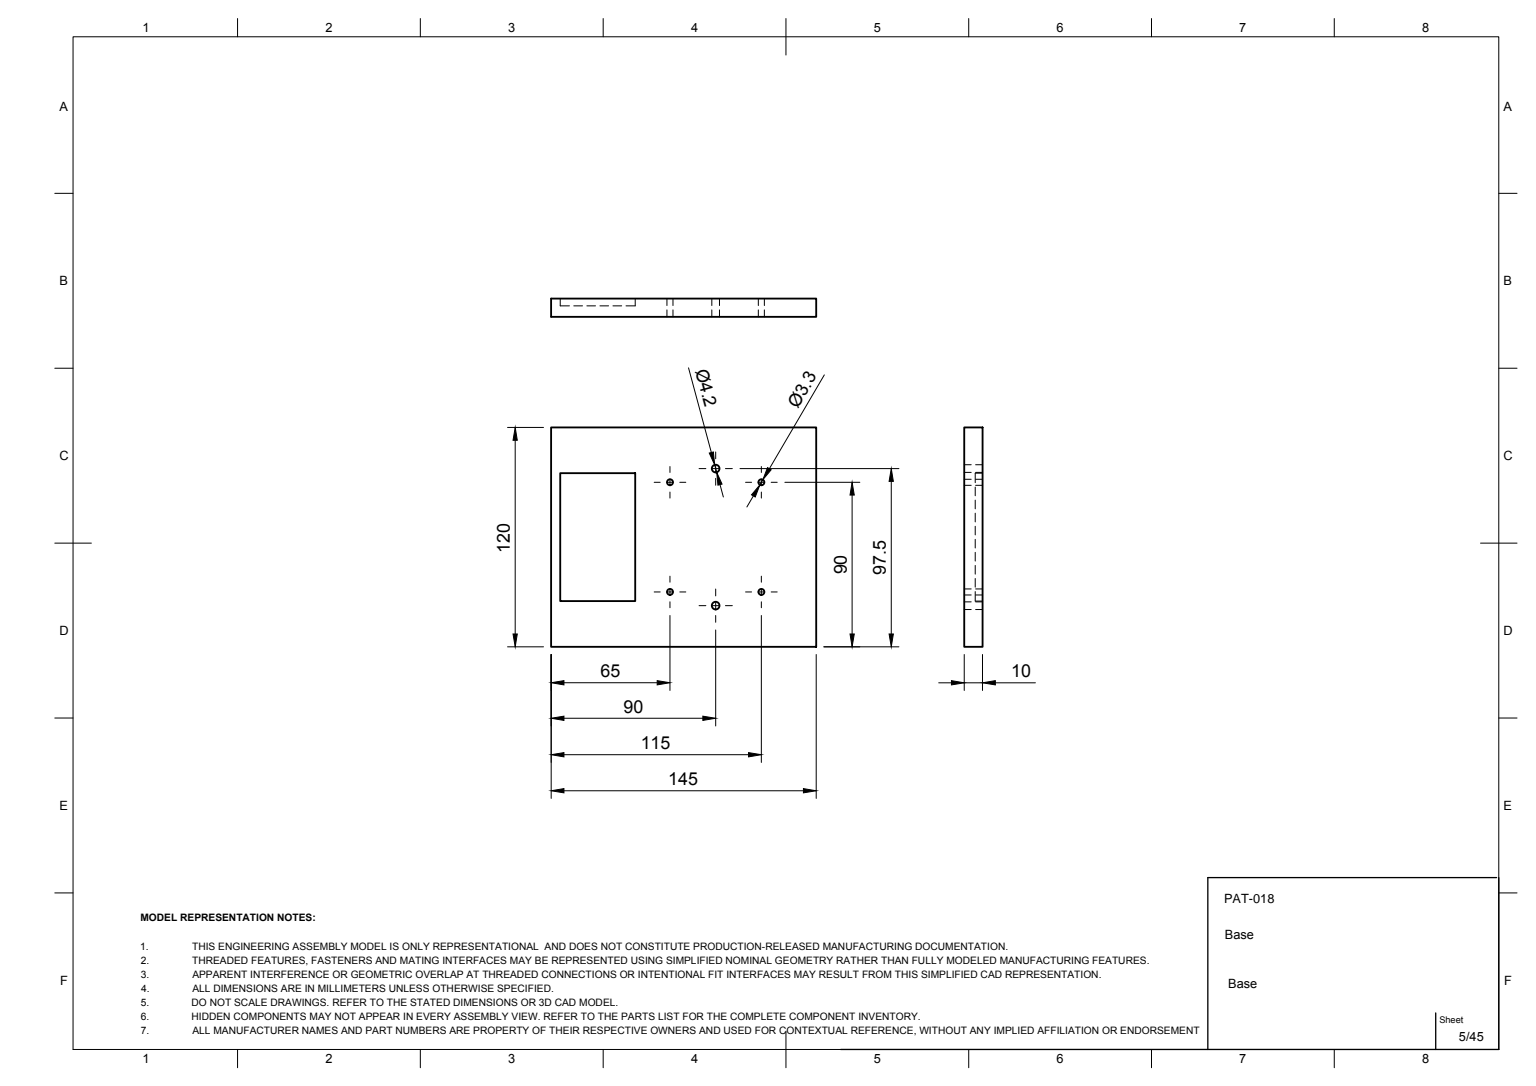
ISO-10303-21;
HEADER;
/* Generated by software containing ST-Developer
 * from STEP Tools, Inc. (www.steptools.com) 
 */

FILE_DESCRIPTION(
/* description */ ('Cam-driven reciprocating slide'),
/* implementation_level */ '2;1');

FILE_NAME(
/* name */ 'Base.step',
/* time_stamp */ '2026-10-28T03:25:20-07:00',
/* author */ (''),
/* organization */ (''),
/* preprocessor_version */ 'ST-DEVELOPER v20.2',
/* originating_system */ 'Autodesk Translation Framework v15.17.0.0',
/* authorisation */ '');

FILE_SCHEMA (('AUTOMOTIVE_DESIGN { 1 0 10303 214 3 1 1 }'));
ENDSEC;

DATA;
#10=MECHANICAL_DESIGN_GEOMETRIC_PRESENTATION_REPRESENTATION('',(#422),#13277);
#348=SHAPE_REPRESENTATION_RELATIONSHIP('SRR','None',#13441,#385);
#385=ADVANCED_BREP_SHAPE_REPRESENTATION('',(#466),#13236);
#422=STYLED_ITEM('',(#13699),#466);
#466=MANIFOLD_SOLID_BREP('Body1',#6398);
#507=FACE_BOUND('',#1296,.T.);
#508=FACE_BOUND('',#1297,.T.);
#509=FACE_BOUND('',#1298,.T.);
#510=FACE_BOUND('',#1299,.T.);
#511=FACE_BOUND('',#1300,.T.);
#512=FACE_BOUND('',#1301,.T.);
#513=FACE_BOUND('',#1302,.T.);
#514=FACE_BOUND('',#1304,.T.);
#515=FACE_BOUND('',#1305,.T.);
#516=FACE_BOUND('',#1306,.T.);
#517=FACE_BOUND('',#1307,.T.);
#518=FACE_BOUND('',#1308,.T.);
#519=FACE_BOUND('',#1309,.T.);
#681=PLANE('',#6874);
#682=PLANE('',#6875);
#683=PLANE('',#6876);
#684=PLANE('',#6877);
#685=PLANE('',#6878);
#686=PLANE('',#6879);
#687=PLANE('',#6880);
#688=PLANE('',#6881);
#689=PLANE('',#6882);
#690=PLANE('',#6883);
#691=PLANE('',#6884);
#901=FACE_OUTER_BOUND('',#1280,.T.);
#902=FACE_OUTER_BOUND('',#1281,.T.);
#903=FACE_OUTER_BOUND('',#1282,.T.);
#904=FACE_OUTER_BOUND('',#1283,.T.);
#905=FACE_OUTER_BOUND('',#1284,.T.);
#906=FACE_OUTER_BOUND('',#1285,.T.);
#907=FACE_OUTER_BOUND('',#1286,.T.);
#908=FACE_OUTER_BOUND('',#1287,.T.);
#909=FACE_OUTER_BOUND('',#1288,.T.);
#910=FACE_OUTER_BOUND('',#1289,.T.);
#911=FACE_OUTER_BOUND('',#1290,.T.);
#912=FACE_OUTER_BOUND('',#1291,.T.);
#913=FACE_OUTER_BOUND('',#1292,.T.);
#914=FACE_OUTER_BOUND('',#1293,.T.);
#915=FACE_OUTER_BOUND('',#1294,.T.);
#916=FACE_OUTER_BOUND('',#1295,.T.);
#917=FACE_OUTER_BOUND('',#1303,.T.);
#1280=EDGE_LOOP('',(#4336,#4337,#4338,#4339));
#1281=EDGE_LOOP('',(#4340,#4341,#4342,#4343));
#1282=EDGE_LOOP('',(#4344,#4345,#4346,#4347));
#1283=EDGE_LOOP('',(#4348,#4349,#4350,#4351));
#1284=EDGE_LOOP('',(#4352,#4353,#4354,#4355));
#1285=EDGE_LOOP('',(#4356,#4357,#4358,#4359));
#1286=EDGE_LOOP('',(#4360,#4361,#4362,#4363));
#1287=EDGE_LOOP('',(#4364,#4365,#4366,#4367));
#1288=EDGE_LOOP('',(#4368,#4369,#4370,#4371));
#1289=EDGE_LOOP('',(#4372,#4373,#4374,#4375));
#1290=EDGE_LOOP('',(#4376,#4377,#4378,#4379));
#1291=EDGE_LOOP('',(#4380,#4381,#4382,#4383));
#1292=EDGE_LOOP('',(#4384,#4385,#4386,#4387));
#1293=EDGE_LOOP('',(#4388,#4389,#4390,#4391));
#1294=EDGE_LOOP('',(#4392,#4393,#4394,#4395));
#1295=EDGE_LOOP('',(#4396,#4397,#4398,#4399));
#1296=EDGE_LOOP('',(#4400));
#1297=EDGE_LOOP('',(#4401));
#1298=EDGE_LOOP('',(#4402));
#1299=EDGE_LOOP('',(#4403));
#1300=EDGE_LOOP('',(#4404));
#1301=EDGE_LOOP('',(#4405));
#1302=EDGE_LOOP('',(#4406,#4407,#4408,#4409));
#1303=EDGE_LOOP('',(#4410,#4411,#4412,#4413));
#1304=EDGE_LOOP('',(#4414));
#1305=EDGE_LOOP('',(#4415));
#1306=EDGE_LOOP('',(#4416));
#1307=EDGE_LOOP('',(#4417));
#1308=EDGE_LOOP('',(#4418));
#1309=EDGE_LOOP('',(#4419));
#1833=LINE('',#9747,#2272);
#1834=LINE('',#9753,#2273);
#1835=LINE('',#9759,#2274);
#1836=LINE('',#9765,#2275);
#1837=LINE('',#9771,#2276);
#1838=LINE('',#9777,#2277);
#1839=LINE('',#9782,#2278);
#1840=LINE('',#9784,#2279);
#1841=LINE('',#9786,#2280);
#1842=LINE('',#9787,#2281);
#1843=LINE('',#9790,#2282);
#1844=LINE('',#9792,#2283);
#1845=LINE('',#9793,#2284);
#1846=LINE('',#9796,#2285);
#1847=LINE('',#9798,#2286);
#1848=LINE('',#9799,#2287);
#1849=LINE('',#9801,#2288);
#1850=LINE('',#9802,#2289);
#1851=LINE('',#9807,#2290);
#1852=LINE('',#9809,#2291);
#1853=LINE('',#9811,#2292);
#1854=LINE('',#9812,#2293);
#1855=LINE('',#9815,#2294);
#1856=LINE('',#9817,#2295);
#1857=LINE('',#9818,#2296);
#1858=LINE('',#9821,#2297);
#1859=LINE('',#9823,#2298);
#1860=LINE('',#9824,#2299);
#1861=LINE('',#9826,#2300);
#1862=LINE('',#9827,#2301);
#2272=VECTOR('',#7679,0.21);
#2273=VECTOR('',#7686,0.21);
#2274=VECTOR('',#7693,0.165);
#2275=VECTOR('',#7700,0.165);
#2276=VECTOR('',#7707,0.165);
#2277=VECTOR('',#7714,0.165);
#2278=VECTOR('',#7719,1.);
#2279=VECTOR('',#7720,1.);
#2280=VECTOR('',#7721,1.);
#2281=VECTOR('',#7722,1.);
#2282=VECTOR('',#7725,1.);
#2283=VECTOR('',#7726,1.);
#2284=VECTOR('',#7727,1.);
#2285=VECTOR('',#7730,1.);
#2286=VECTOR('',#7731,1.);
#2287=VECTOR('',#7732,1.);
#2288=VECTOR('',#7735,1.);
#2289=VECTOR('',#7736,1.);
#2290=VECTOR('',#7741,1.);
#2291=VECTOR('',#7742,1.);
#2292=VECTOR('',#7743,1.);
#2293=VECTOR('',#7744,1.);
#2294=VECTOR('',#7747,1.);
#2295=VECTOR('',#7748,1.);
#2296=VECTOR('',#7749,1.);
#2297=VECTOR('',#7752,1.);
#2298=VECTOR('',#7753,1.);
#2299=VECTOR('',#7754,1.);
#2300=VECTOR('',#7757,1.);
#2301=VECTOR('',#7758,1.);
#2711=CIRCLE('',#6857,0.21);
#2712=CIRCLE('',#6858,0.21);
#2713=CIRCLE('',#6860,0.21);
#2714=CIRCLE('',#6861,0.21);
#2715=CIRCLE('',#6863,0.165);
#2716=CIRCLE('',#6864,0.165);
#2717=CIRCLE('',#6866,0.165);
#2718=CIRCLE('',#6867,0.165);
#2719=CIRCLE('',#6869,0.165);
#2720=CIRCLE('',#6870,0.165);
#2721=CIRCLE('',#6872,0.165);
#2722=CIRCLE('',#6873,0.165);
#3035=VERTEX_POINT('',#9744);
#3036=VERTEX_POINT('',#9746);
#3037=VERTEX_POINT('',#9750);
#3038=VERTEX_POINT('',#9752);
#3039=VERTEX_POINT('',#9756);
#3040=VERTEX_POINT('',#9758);
#3041=VERTEX_POINT('',#9762);
#3042=VERTEX_POINT('',#9764);
#3043=VERTEX_POINT('',#9768);
#3044=VERTEX_POINT('',#9770);
#3045=VERTEX_POINT('',#9774);
#3046=VERTEX_POINT('',#9776);
#3047=VERTEX_POINT('',#9780);
#3048=VERTEX_POINT('',#9781);
#3049=VERTEX_POINT('',#9783);
#3050=VERTEX_POINT('',#9785);
#3051=VERTEX_POINT('',#9789);
#3052=VERTEX_POINT('',#9791);
#3053=VERTEX_POINT('',#9795);
#3054=VERTEX_POINT('',#9797);
#3055=VERTEX_POINT('',#9805);
#3056=VERTEX_POINT('',#9806);
#3057=VERTEX_POINT('',#9808);
#3058=VERTEX_POINT('',#9810);
#3059=VERTEX_POINT('',#9814);
#3060=VERTEX_POINT('',#9816);
#3061=VERTEX_POINT('',#9820);
#3062=VERTEX_POINT('',#9822);
#3558=EDGE_CURVE('',#3035,#3035,#2711,.T.);
#3559=EDGE_CURVE('',#3035,#3036,#1833,.T.);
#3560=EDGE_CURVE('',#3036,#3036,#2712,.T.);
#3561=EDGE_CURVE('',#3037,#3037,#2713,.T.);
#3562=EDGE_CURVE('',#3037,#3038,#1834,.T.);
#3563=EDGE_CURVE('',#3038,#3038,#2714,.T.);
#3564=EDGE_CURVE('',#3039,#3039,#2715,.T.);
#3565=EDGE_CURVE('',#3039,#3040,#1835,.T.);
#3566=EDGE_CURVE('',#3040,#3040,#2716,.T.);
#3567=EDGE_CURVE('',#3041,#3041,#2717,.T.);
#3568=EDGE_CURVE('',#3041,#3042,#1836,.T.);
#3569=EDGE_CURVE('',#3042,#3042,#2718,.T.);
#3570=EDGE_CURVE('',#3043,#3043,#2719,.T.);
#3571=EDGE_CURVE('',#3043,#3044,#1837,.T.);
#3572=EDGE_CURVE('',#3044,#3044,#2720,.T.);
#3573=EDGE_CURVE('',#3045,#3045,#2721,.T.);
#3574=EDGE_CURVE('',#3045,#3046,#1838,.T.);
#3575=EDGE_CURVE('',#3046,#3046,#2722,.T.);
#3576=EDGE_CURVE('',#3047,#3048,#1839,.T.);
#3577=EDGE_CURVE('',#3049,#3047,#1840,.T.);
#3578=EDGE_CURVE('',#3050,#3049,#1841,.T.);
#3579=EDGE_CURVE('',#3050,#3048,#1842,.T.);
#3580=EDGE_CURVE('',#3048,#3051,#1843,.T.);
#3581=EDGE_CURVE('',#3052,#3050,#1844,.T.);
#3582=EDGE_CURVE('',#3052,#3051,#1845,.T.);
#3583=EDGE_CURVE('',#3051,#3053,#1846,.T.);
#3584=EDGE_CURVE('',#3054,#3052,#1847,.T.);
#3585=EDGE_CURVE('',#3054,#3053,#1848,.T.);
#3586=EDGE_CURVE('',#3053,#3047,#1849,.T.);
#3587=EDGE_CURVE('',#3049,#3054,#1850,.T.);
#3588=EDGE_CURVE('',#3055,#3056,#1851,.T.);
#3589=EDGE_CURVE('',#3056,#3057,#1852,.T.);
#3590=EDGE_CURVE('',#3058,#3057,#1853,.T.);
#3591=EDGE_CURVE('',#3055,#3058,#1854,.T.);
#3592=EDGE_CURVE('',#3059,#3055,#1855,.T.);
#3593=EDGE_CURVE('',#3060,#3058,#1856,.T.);
#3594=EDGE_CURVE('',#3059,#3060,#1857,.T.);
#3595=EDGE_CURVE('',#3061,#3059,#1858,.T.);
#3596=EDGE_CURVE('',#3062,#3060,#1859,.T.);
#3597=EDGE_CURVE('',#3061,#3062,#1860,.T.);
#3598=EDGE_CURVE('',#3056,#3061,#1861,.T.);
#3599=EDGE_CURVE('',#3057,#3062,#1862,.T.);
#4336=ORIENTED_EDGE('',*,*,#3558,.F.);
#4337=ORIENTED_EDGE('',*,*,#3559,.T.);
#4338=ORIENTED_EDGE('',*,*,#3560,.F.);
#4339=ORIENTED_EDGE('',*,*,#3559,.F.);
#4340=ORIENTED_EDGE('',*,*,#3561,.F.);
#4341=ORIENTED_EDGE('',*,*,#3562,.T.);
#4342=ORIENTED_EDGE('',*,*,#3563,.F.);
#4343=ORIENTED_EDGE('',*,*,#3562,.F.);
#4344=ORIENTED_EDGE('',*,*,#3564,.F.);
#4345=ORIENTED_EDGE('',*,*,#3565,.T.);
#4346=ORIENTED_EDGE('',*,*,#3566,.F.);
#4347=ORIENTED_EDGE('',*,*,#3565,.F.);
#4348=ORIENTED_EDGE('',*,*,#3567,.F.);
#4349=ORIENTED_EDGE('',*,*,#3568,.T.);
#4350=ORIENTED_EDGE('',*,*,#3569,.F.);
#4351=ORIENTED_EDGE('',*,*,#3568,.F.);
#4352=ORIENTED_EDGE('',*,*,#3570,.F.);
#4353=ORIENTED_EDGE('',*,*,#3571,.T.);
#4354=ORIENTED_EDGE('',*,*,#3572,.F.);
#4355=ORIENTED_EDGE('',*,*,#3571,.F.);
#4356=ORIENTED_EDGE('',*,*,#3573,.F.);
#4357=ORIENTED_EDGE('',*,*,#3574,.T.);
#4358=ORIENTED_EDGE('',*,*,#3575,.F.);
#4359=ORIENTED_EDGE('',*,*,#3574,.F.);
#4360=ORIENTED_EDGE('',*,*,#3576,.F.);
#4361=ORIENTED_EDGE('',*,*,#3577,.F.);
#4362=ORIENTED_EDGE('',*,*,#3578,.F.);
#4363=ORIENTED_EDGE('',*,*,#3579,.T.);
#4364=ORIENTED_EDGE('',*,*,#3580,.F.);
#4365=ORIENTED_EDGE('',*,*,#3579,.F.);
#4366=ORIENTED_EDGE('',*,*,#3581,.F.);
#4367=ORIENTED_EDGE('',*,*,#3582,.T.);
#4368=ORIENTED_EDGE('',*,*,#3583,.F.);
#4369=ORIENTED_EDGE('',*,*,#3582,.F.);
#4370=ORIENTED_EDGE('',*,*,#3584,.F.);
#4371=ORIENTED_EDGE('',*,*,#3585,.T.);
#4372=ORIENTED_EDGE('',*,*,#3586,.F.);
#4373=ORIENTED_EDGE('',*,*,#3585,.F.);
#4374=ORIENTED_EDGE('',*,*,#3587,.F.);
#4375=ORIENTED_EDGE('',*,*,#3577,.T.);
#4376=ORIENTED_EDGE('',*,*,#3581,.T.);
#4377=ORIENTED_EDGE('',*,*,#3578,.T.);
#4378=ORIENTED_EDGE('',*,*,#3587,.T.);
#4379=ORIENTED_EDGE('',*,*,#3584,.T.);
#4380=ORIENTED_EDGE('',*,*,#3588,.T.);
#4381=ORIENTED_EDGE('',*,*,#3589,.T.);
#4382=ORIENTED_EDGE('',*,*,#3590,.F.);
#4383=ORIENTED_EDGE('',*,*,#3591,.F.);
#4384=ORIENTED_EDGE('',*,*,#3592,.T.);
#4385=ORIENTED_EDGE('',*,*,#3591,.T.);
#4386=ORIENTED_EDGE('',*,*,#3593,.F.);
#4387=ORIENTED_EDGE('',*,*,#3594,.F.);
#4388=ORIENTED_EDGE('',*,*,#3595,.T.);
#4389=ORIENTED_EDGE('',*,*,#3594,.T.);
#4390=ORIENTED_EDGE('',*,*,#3596,.F.);
#4391=ORIENTED_EDGE('',*,*,#3597,.F.);
#4392=ORIENTED_EDGE('',*,*,#3598,.T.);
#4393=ORIENTED_EDGE('',*,*,#3597,.T.);
#4394=ORIENTED_EDGE('',*,*,#3599,.F.);
#4395=ORIENTED_EDGE('',*,*,#3589,.F.);
#4396=ORIENTED_EDGE('',*,*,#3599,.T.);
#4397=ORIENTED_EDGE('',*,*,#3596,.T.);
#4398=ORIENTED_EDGE('',*,*,#3593,.T.);
#4399=ORIENTED_EDGE('',*,*,#3590,.T.);
#4400=ORIENTED_EDGE('',*,*,#3560,.T.);
#4401=ORIENTED_EDGE('',*,*,#3563,.T.);
#4402=ORIENTED_EDGE('',*,*,#3566,.T.);
#4403=ORIENTED_EDGE('',*,*,#3569,.T.);
#4404=ORIENTED_EDGE('',*,*,#3572,.T.);
#4405=ORIENTED_EDGE('',*,*,#3575,.T.);
#4406=ORIENTED_EDGE('',*,*,#3583,.T.);
#4407=ORIENTED_EDGE('',*,*,#3586,.T.);
#4408=ORIENTED_EDGE('',*,*,#3576,.T.);
#4409=ORIENTED_EDGE('',*,*,#3580,.T.);
#4410=ORIENTED_EDGE('',*,*,#3598,.F.);
#4411=ORIENTED_EDGE('',*,*,#3588,.F.);
#4412=ORIENTED_EDGE('',*,*,#3592,.F.);
#4413=ORIENTED_EDGE('',*,*,#3595,.F.);
#4414=ORIENTED_EDGE('',*,*,#3558,.T.);
#4415=ORIENTED_EDGE('',*,*,#3561,.T.);
#4416=ORIENTED_EDGE('',*,*,#3564,.T.);
#4417=ORIENTED_EDGE('',*,*,#3567,.T.);
#4418=ORIENTED_EDGE('',*,*,#3570,.T.);
#4419=ORIENTED_EDGE('',*,*,#3573,.T.);
#5892=CYLINDRICAL_SURFACE('',#6856,0.21);
#5893=CYLINDRICAL_SURFACE('',#6859,0.21);
#5894=CYLINDRICAL_SURFACE('',#6862,0.165);
#5895=CYLINDRICAL_SURFACE('',#6865,0.165);
#5896=CYLINDRICAL_SURFACE('',#6868,0.165);
#5897=CYLINDRICAL_SURFACE('',#6871,0.165);
#6019=ADVANCED_FACE('',(#901),#5892,.F.);
#6020=ADVANCED_FACE('',(#902),#5893,.F.);
#6021=ADVANCED_FACE('',(#903),#5894,.F.);
#6022=ADVANCED_FACE('',(#904),#5895,.F.);
#6023=ADVANCED_FACE('',(#905),#5896,.F.);
#6024=ADVANCED_FACE('',(#906),#5897,.F.);
#6025=ADVANCED_FACE('',(#907),#681,.F.);
#6026=ADVANCED_FACE('',(#908),#682,.F.);
#6027=ADVANCED_FACE('',(#909),#683,.F.);
#6028=ADVANCED_FACE('',(#910),#684,.F.);
#6029=ADVANCED_FACE('',(#911),#685,.T.);
#6030=ADVANCED_FACE('',(#912),#686,.T.);
#6031=ADVANCED_FACE('',(#913),#687,.T.);
#6032=ADVANCED_FACE('',(#914),#688,.T.);
#6033=ADVANCED_FACE('',(#915),#689,.T.);
#6034=ADVANCED_FACE('',(#916,#507,#508,#509,#510,#511,#512,#513),#690,.T.);
#6035=ADVANCED_FACE('',(#917,#514,#515,#516,#517,#518,#519),#691,.F.);
#6398=CLOSED_SHELL('',(#6019,#6020,#6021,#6022,#6023,#6024,#6025,#6026,
#6027,#6028,#6029,#6030,#6031,#6032,#6033,#6034,#6035));
#6855=AXIS2_PLACEMENT_3D('',#9742,#7673,#7674);
#6856=AXIS2_PLACEMENT_3D('',#9743,#7675,#7676);
#6857=AXIS2_PLACEMENT_3D('',#9745,#7677,#7678);
#6858=AXIS2_PLACEMENT_3D('',#9748,#7680,#7681);
#6859=AXIS2_PLACEMENT_3D('',#9749,#7682,#7683);
#6860=AXIS2_PLACEMENT_3D('',#9751,#7684,#7685);
#6861=AXIS2_PLACEMENT_3D('',#9754,#7687,#7688);
#6862=AXIS2_PLACEMENT_3D('',#9755,#7689,#7690);
#6863=AXIS2_PLACEMENT_3D('',#9757,#7691,#7692);
#6864=AXIS2_PLACEMENT_3D('',#9760,#7694,#7695);
#6865=AXIS2_PLACEMENT_3D('',#9761,#7696,#7697);
#6866=AXIS2_PLACEMENT_3D('',#9763,#7698,#7699);
#6867=AXIS2_PLACEMENT_3D('',#9766,#7701,#7702);
#6868=AXIS2_PLACEMENT_3D('',#9767,#7703,#7704);
#6869=AXIS2_PLACEMENT_3D('',#9769,#7705,#7706);
#6870=AXIS2_PLACEMENT_3D('',#9772,#7708,#7709);
#6871=AXIS2_PLACEMENT_3D('',#9773,#7710,#7711);
#6872=AXIS2_PLACEMENT_3D('',#9775,#7712,#7713);
#6873=AXIS2_PLACEMENT_3D('',#9778,#7715,#7716);
#6874=AXIS2_PLACEMENT_3D('',#9779,#7717,#7718);
#6875=AXIS2_PLACEMENT_3D('',#9788,#7723,#7724);
#6876=AXIS2_PLACEMENT_3D('',#9794,#7728,#7729);
#6877=AXIS2_PLACEMENT_3D('',#9800,#7733,#7734);
#6878=AXIS2_PLACEMENT_3D('',#9803,#7737,#7738);
#6879=AXIS2_PLACEMENT_3D('',#9804,#7739,#7740);
#6880=AXIS2_PLACEMENT_3D('',#9813,#7745,#7746);
#6881=AXIS2_PLACEMENT_3D('',#9819,#7750,#7751);
#6882=AXIS2_PLACEMENT_3D('',#9825,#7755,#7756);
#6883=AXIS2_PLACEMENT_3D('',#9828,#7759,#7760);
#6884=AXIS2_PLACEMENT_3D('',#9829,#7761,#7762);
#7673=DIRECTION('axis',(0.,0.,1.));
#7674=DIRECTION('refdir',(1.,0.,0.));
#7675=DIRECTION('center_axis',(0.,0.,1.));
#7676=DIRECTION('ref_axis',(1.,0.,0.));
#7677=DIRECTION('center_axis',(0.,0.,1.));
#7678=DIRECTION('ref_axis',(1.,0.,0.));
#7679=DIRECTION('',(0.,0.,1.));
#7680=DIRECTION('center_axis',(0.,0.,-1.));
#7681=DIRECTION('ref_axis',(1.,0.,0.));
#7682=DIRECTION('center_axis',(0.,0.,1.));
#7683=DIRECTION('ref_axis',(1.,0.,0.));
#7684=DIRECTION('center_axis',(0.,0.,1.));
#7685=DIRECTION('ref_axis',(1.,0.,0.));
#7686=DIRECTION('',(0.,0.,1.));
#7687=DIRECTION('center_axis',(0.,0.,-1.));
#7688=DIRECTION('ref_axis',(1.,0.,0.));
#7689=DIRECTION('center_axis',(0.,0.,1.));
#7690=DIRECTION('ref_axis',(1.,0.,0.));
#7691=DIRECTION('center_axis',(0.,0.,1.));
#7692=DIRECTION('ref_axis',(1.,0.,0.));
#7693=DIRECTION('',(0.,0.,1.));
#7694=DIRECTION('center_axis',(0.,0.,-1.));
#7695=DIRECTION('ref_axis',(1.,0.,0.));
#7696=DIRECTION('center_axis',(0.,0.,1.));
#7697=DIRECTION('ref_axis',(1.,0.,0.));
#7698=DIRECTION('center_axis',(0.,0.,1.));
#7699=DIRECTION('ref_axis',(1.,0.,0.));
#7700=DIRECTION('',(0.,0.,1.));
#7701=DIRECTION('center_axis',(0.,0.,-1.));
#7702=DIRECTION('ref_axis',(1.,0.,0.));
#7703=DIRECTION('center_axis',(0.,0.,1.));
#7704=DIRECTION('ref_axis',(1.,0.,0.));
#7705=DIRECTION('center_axis',(0.,0.,1.));
#7706=DIRECTION('ref_axis',(1.,0.,0.));
#7707=DIRECTION('',(0.,0.,1.));
#7708=DIRECTION('center_axis',(0.,0.,-1.));
#7709=DIRECTION('ref_axis',(1.,0.,0.));
#7710=DIRECTION('center_axis',(0.,0.,1.));
#7711=DIRECTION('ref_axis',(1.,0.,0.));
#7712=DIRECTION('center_axis',(0.,0.,1.));
#7713=DIRECTION('ref_axis',(1.,0.,0.));
#7714=DIRECTION('',(0.,0.,1.));
#7715=DIRECTION('center_axis',(0.,0.,-1.));
#7716=DIRECTION('ref_axis',(1.,0.,0.));
#7717=DIRECTION('center_axis',(0.,-1.,0.));
#7718=DIRECTION('ref_axis',(1.,0.,0.));
#7719=DIRECTION('',(-1.,0.,0.));
#7720=DIRECTION('',(0.,0.,1.));
#7721=DIRECTION('',(1.,0.,0.));
#7722=DIRECTION('',(0.,0.,1.));
#7723=DIRECTION('center_axis',(-1.,0.,0.));
#7724=DIRECTION('ref_axis',(0.,-1.,0.));
#7725=DIRECTION('',(0.,1.,0.));
#7726=DIRECTION('',(0.,-1.,0.));
#7727=DIRECTION('',(0.,0.,1.));
#7728=DIRECTION('center_axis',(0.,1.,0.));
#7729=DIRECTION('ref_axis',(-1.,0.,0.));
#7730=DIRECTION('',(1.,0.,0.));
#7731=DIRECTION('',(-1.,0.,0.));
#7732=DIRECTION('',(0.,0.,1.));
#7733=DIRECTION('center_axis',(1.,0.,0.));
#7734=DIRECTION('ref_axis',(0.,1.,0.));
#7735=DIRECTION('',(0.,-1.,0.));
#7736=DIRECTION('',(0.,1.,0.));
#7737=DIRECTION('center_axis',(0.,0.,1.));
#7738=DIRECTION('ref_axis',(1.,0.,0.));
#7739=DIRECTION('center_axis',(0.,1.,0.));
#7740=DIRECTION('ref_axis',(-1.,0.,0.));
#7741=DIRECTION('',(-1.,0.,0.));
#7742=DIRECTION('',(0.,0.,1.));
#7743=DIRECTION('',(-1.,0.,0.));
#7744=DIRECTION('',(0.,0.,1.));
#7745=DIRECTION('center_axis',(1.,0.,0.));
#7746=DIRECTION('ref_axis',(0.,1.,0.));
#7747=DIRECTION('',(0.,1.,0.));
#7748=DIRECTION('',(0.,1.,0.));
#7749=DIRECTION('',(0.,0.,1.));
#7750=DIRECTION('center_axis',(0.,-1.,0.));
#7751=DIRECTION('ref_axis',(1.,0.,0.));
#7752=DIRECTION('',(1.,0.,0.));
#7753=DIRECTION('',(1.,0.,0.));
#7754=DIRECTION('',(0.,0.,1.));
#7755=DIRECTION('center_axis',(-1.,0.,0.));
#7756=DIRECTION('ref_axis',(0.,-1.,0.));
#7757=DIRECTION('',(0.,-1.,0.));
#7758=DIRECTION('',(0.,-1.,0.));
#7759=DIRECTION('center_axis',(0.,0.,1.));
#7760=DIRECTION('ref_axis',(1.,0.,0.));
#7761=DIRECTION('center_axis',(0.,0.,1.));
#7762=DIRECTION('ref_axis',(1.,0.,0.));
#9742=CARTESIAN_POINT('',(0.,0.,0.));
#9743=CARTESIAN_POINT('Origin',(3.75,0.,-0.1));
#9744=CARTESIAN_POINT('',(3.54,-2.57175827820944E-17,0.));
#9745=CARTESIAN_POINT('Origin',(3.75,0.,0.));
#9746=CARTESIAN_POINT('',(3.54,2.57175827820944E-17,1.));
#9747=CARTESIAN_POINT('',(3.54,-2.57175827820944E-17,-0.1));
#9748=CARTESIAN_POINT('Origin',(3.75,0.,1.));
#9749=CARTESIAN_POINT('Origin',(-3.75,0.,-0.1));
#9750=CARTESIAN_POINT('',(-3.96,-2.57175827820944E-17,0.));
#9751=CARTESIAN_POINT('Origin',(-3.75,0.,0.));
#9752=CARTESIAN_POINT('',(-3.96,2.57175827820944E-17,1.));
#9753=CARTESIAN_POINT('',(-3.96,-2.57175827820944E-17,-0.1));
#9754=CARTESIAN_POINT('Origin',(-3.75,0.,1.));
#9755=CARTESIAN_POINT('Origin',(-3.,2.5,-0.1));
#9756=CARTESIAN_POINT('',(-3.165,2.5,0.));
#9757=CARTESIAN_POINT('Origin',(-3.,2.5,0.));
#9758=CARTESIAN_POINT('',(-3.165,2.5,1.));
#9759=CARTESIAN_POINT('',(-3.165,2.5,-0.1));
#9760=CARTESIAN_POINT('Origin',(-3.,2.5,1.));
#9761=CARTESIAN_POINT('Origin',(3.,2.5,-0.1));
#9762=CARTESIAN_POINT('',(2.835,2.5,0.));
#9763=CARTESIAN_POINT('Origin',(3.,2.5,0.));
#9764=CARTESIAN_POINT('',(2.835,2.5,1.));
#9765=CARTESIAN_POINT('',(2.835,2.5,-0.1));
#9766=CARTESIAN_POINT('Origin',(3.,2.5,1.));
#9767=CARTESIAN_POINT('Origin',(-3.,-2.5,-0.1));
#9768=CARTESIAN_POINT('',(-3.165,-2.5,0.));
#9769=CARTESIAN_POINT('Origin',(-3.,-2.5,0.));
#9770=CARTESIAN_POINT('',(-3.165,-2.5,1.));
#9771=CARTESIAN_POINT('',(-3.165,-2.5,-0.1));
#9772=CARTESIAN_POINT('Origin',(-3.,-2.5,1.));
#9773=CARTESIAN_POINT('Origin',(3.,-2.5,-0.1));
#9774=CARTESIAN_POINT('',(2.835,-2.5,0.));
#9775=CARTESIAN_POINT('Origin',(3.,-2.5,0.));
#9776=CARTESIAN_POINT('',(2.835,-2.5,1.));
#9777=CARTESIAN_POINT('',(2.835,-2.5,-0.1));
#9778=CARTESIAN_POINT('Origin',(3.,-2.5,1.));
#9779=CARTESIAN_POINT('Origin',(-3.5,4.4,0.6));
#9780=CARTESIAN_POINT('',(3.5,4.4,1.));
#9781=CARTESIAN_POINT('',(-3.5,4.4,1.));
#9782=CARTESIAN_POINT('',(-1.75,4.4,1.));
#9783=CARTESIAN_POINT('',(3.5,4.4,0.6));
#9784=CARTESIAN_POINT('',(3.5,4.4,0.6));
#9785=CARTESIAN_POINT('',(-3.5,4.4,0.6));
#9786=CARTESIAN_POINT('',(-3.5,4.4,0.6));
#9787=CARTESIAN_POINT('',(-3.5,4.4,0.6));
#9788=CARTESIAN_POINT('Origin',(-3.5,8.5,0.6));
#9789=CARTESIAN_POINT('',(-3.5,8.5,1.));
#9790=CARTESIAN_POINT('',(-3.5,5.125,1.));
#9791=CARTESIAN_POINT('',(-3.5,8.5,0.6));
#9792=CARTESIAN_POINT('',(-3.5,8.5,0.6));
#9793=CARTESIAN_POINT('',(-3.5,8.5,0.6));
#9794=CARTESIAN_POINT('Origin',(3.5,8.5,0.6));
#9795=CARTESIAN_POINT('',(3.5,8.5,1.));
#9796=CARTESIAN_POINT('',(1.75,8.5,1.));
#9797=CARTESIAN_POINT('',(3.5,8.5,0.6));
#9798=CARTESIAN_POINT('',(3.5,8.5,0.6));
#9799=CARTESIAN_POINT('',(3.5,8.5,0.6));
#9800=CARTESIAN_POINT('Origin',(3.5,4.4,0.6));
#9801=CARTESIAN_POINT('',(3.5,3.075,1.));
#9802=CARTESIAN_POINT('',(3.5,4.4,0.6));
#9803=CARTESIAN_POINT('Origin',(0.,6.45,0.6));
#9804=CARTESIAN_POINT('Origin',(6.,9.,0.));
#9805=CARTESIAN_POINT('',(6.,9.,0.));
#9806=CARTESIAN_POINT('',(-6.,9.,0.));
#9807=CARTESIAN_POINT('',(6.,9.,0.));
#9808=CARTESIAN_POINT('',(-6.,9.,1.));
#9809=CARTESIAN_POINT('',(-6.,9.,0.));
#9810=CARTESIAN_POINT('',(6.,9.,1.));
#9811=CARTESIAN_POINT('',(6.,9.,1.));
#9812=CARTESIAN_POINT('',(6.,9.,0.));
#9813=CARTESIAN_POINT('Origin',(6.,-5.5,0.));
#9814=CARTESIAN_POINT('',(6.,-5.5,0.));
#9815=CARTESIAN_POINT('',(6.,-5.5,0.));
#9816=CARTESIAN_POINT('',(6.,-5.5,1.));
#9817=CARTESIAN_POINT('',(6.,-5.5,1.));
#9818=CARTESIAN_POINT('',(6.,-5.5,0.));
#9819=CARTESIAN_POINT('Origin',(-6.,-5.5,0.));
#9820=CARTESIAN_POINT('',(-6.,-5.5,0.));
#9821=CARTESIAN_POINT('',(-6.,-5.5,0.));
#9822=CARTESIAN_POINT('',(-6.,-5.5,1.));
#9823=CARTESIAN_POINT('',(-6.,-5.5,1.));
#9824=CARTESIAN_POINT('',(-6.,-5.5,0.));
#9825=CARTESIAN_POINT('Origin',(-6.,9.,0.));
#9826=CARTESIAN_POINT('',(-6.,9.,0.));
#9827=CARTESIAN_POINT('',(-6.,9.,1.));
#9828=CARTESIAN_POINT('Origin',(0.,1.75,1.));
#9829=CARTESIAN_POINT('Origin',(0.,1.75,0.));
#13192=UNCERTAINTY_MEASURE_WITH_UNIT(LENGTH_MEASURE(0.001),#13278,
'DISTANCE_ACCURACY_VALUE',
'Maximum model space distance between geometric entities at asserted c
onnectivities');
#13233=UNCERTAINTY_MEASURE_WITH_UNIT(LENGTH_MEASURE(0.001),#13278,
'DISTANCE_ACCURACY_VALUE',
'Maximum model space distance between geometric entities at asserted c
onnectivities');
#13236=(
GEOMETRIC_REPRESENTATION_CONTEXT(3)
GLOBAL_UNCERTAINTY_ASSIGNED_CONTEXT((#13192))
GLOBAL_UNIT_ASSIGNED_CONTEXT((#13278,#13280,#13281))
REPRESENTATION_CONTEXT('','3D')
);
#13277=(
GEOMETRIC_REPRESENTATION_CONTEXT(3)
GLOBAL_UNCERTAINTY_ASSIGNED_CONTEXT((#13233))
GLOBAL_UNIT_ASSIGNED_CONTEXT((#13278,#13280,#13281))
REPRESENTATION_CONTEXT('','3D')
);
#13278=(
LENGTH_UNIT()
NAMED_UNIT(*)
SI_UNIT(.CENTI.,.METRE.)
);
#13280=(
NAMED_UNIT(*)
PLANE_ANGLE_UNIT()
SI_UNIT($,.RADIAN.)
);
#13281=(
NAMED_UNIT(*)
SI_UNIT($,.STERADIAN.)
SOLID_ANGLE_UNIT()
);
#13284=SHAPE_DEFINITION_REPRESENTATION(#13327,#13441);
#13327=PRODUCT_DEFINITION_SHAPE('',$,#13485);
#13441=SHAPE_REPRESENTATION('',(#6855),#13236);
#13482=PRODUCT_DEFINITION_CONTEXT('part definition',#13613,'design');
#13485=PRODUCT_DEFINITION('Base','Base',#13528,#13482);
#13528=PRODUCT_DEFINITION_FORMATION('',$,#13617);
#13613=APPLICATION_CONTEXT(
'Core Data for Automotive Mechanical Design Process');
#13614=PRODUCT_CONTEXT('part definition',#13613,'mechanical');
#13617=PRODUCT('Base','Base','Base',(#13614));
#13693=COLOUR_RGB('Dark Blue',0.08,0.2,0.34);
#13694=FILL_AREA_STYLE_COLOUR('',#13693);
#13695=FILL_AREA_STYLE('',(#13694));
#13696=SURFACE_STYLE_FILL_AREA(#13695);
#13697=SURFACE_SIDE_STYLE('',(#13696));
#13698=SURFACE_STYLE_USAGE(.BOTH.,#13697);
#13699=PRESENTATION_STYLE_ASSIGNMENT((#13698));
ENDSEC;
END-ISO-10303-21;
